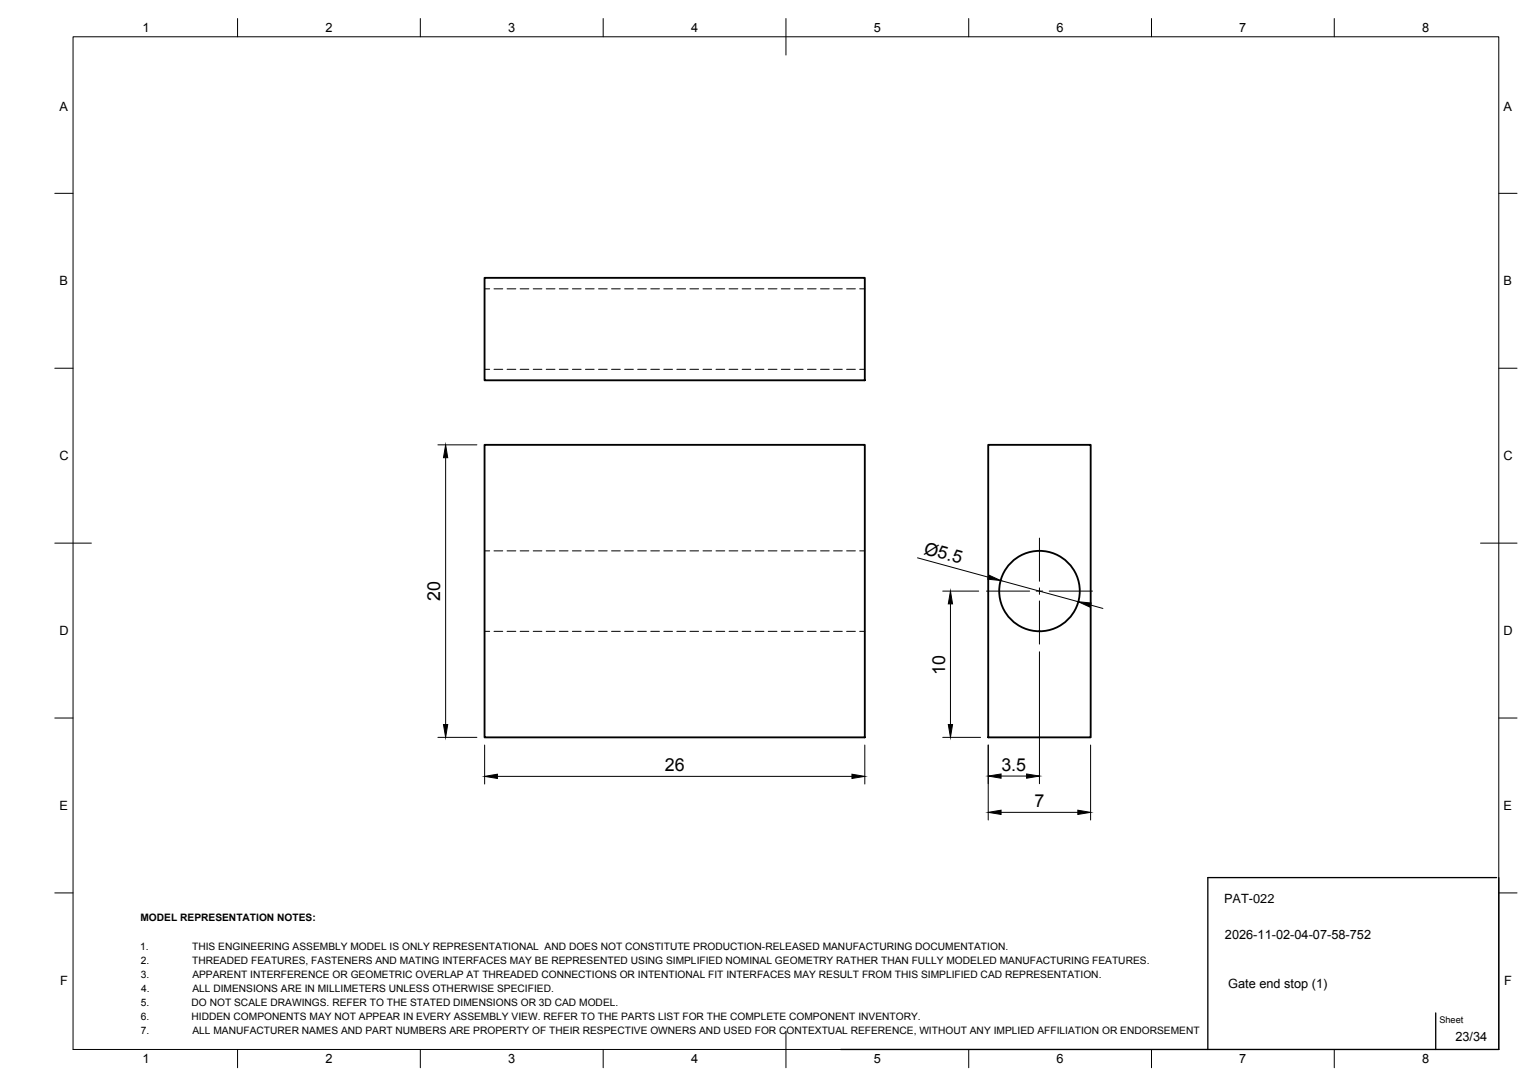
ISO-10303-21;
HEADER;
/* Generated by software containing ST-Developer
 * from STEP Tools, Inc. (www.steptools.com) 
 */

FILE_DESCRIPTION(
/* description */ ('Chute with adjustable gate'),
/* implementation_level */ '2;1');

FILE_NAME(
/* name */ 'Gate end stop (1).step',
/* time_stamp */ '2026-10-27T10:52:28-07:00',
/* author */ (''),
/* organization */ (''),
/* preprocessor_version */ 'ST-DEVELOPER v20.2',
/* originating_system */ 'Autodesk Translation Framework v15.17.0.0',
/* authorisation */ '');

FILE_SCHEMA (('AUTOMOTIVE_DESIGN { 1 0 10303 214 3 1 1 }'));
ENDSEC;

DATA;
#10=MECHANICAL_DESIGN_GEOMETRIC_PRESENTATION_REPRESENTATION('',(#432),#13094);
#368=SHAPE_REPRESENTATION_RELATIONSHIP('SRR','None',#13269,#400);
#400=ADVANCED_BREP_SHAPE_REPRESENTATION('',(#464),#13078);
#432=STYLED_ITEM('',(#13481),#464);
#464=MANIFOLD_SOLID_BREP('Body1',#7615);
#548=FACE_BOUND('',#1583,.T.);
#549=FACE_BOUND('',#1586,.T.);
#728=PLANE('',#8265);
#729=PLANE('',#8266);
#730=PLANE('',#8267);
#731=PLANE('',#8268);
#732=PLANE('',#8269);
#733=PLANE('',#8270);
#1091=FACE_OUTER_BOUND('',#1580,.T.);
#1092=FACE_OUTER_BOUND('',#1581,.T.);
#1093=FACE_OUTER_BOUND('',#1582,.T.);
#1094=FACE_OUTER_BOUND('',#1584,.T.);
#1095=FACE_OUTER_BOUND('',#1585,.T.);
#1096=FACE_OUTER_BOUND('',#1587,.T.);
#1097=FACE_OUTER_BOUND('',#1588,.T.);
#1580=EDGE_LOOP('',(#5972,#5973,#5974,#5975));
#1581=EDGE_LOOP('',(#5976,#5977,#5978,#5979));
#1582=EDGE_LOOP('',(#5980,#5981,#5982,#5983));
#1583=EDGE_LOOP('',(#5984));
#1584=EDGE_LOOP('',(#5985,#5986,#5987,#5988));
#1585=EDGE_LOOP('',(#5989,#5990,#5991,#5992));
#1586=EDGE_LOOP('',(#5993));
#1587=EDGE_LOOP('',(#5994,#5995,#5996,#5997));
#1588=EDGE_LOOP('',(#5998,#5999,#6000,#6001));
#2175=LINE('',#11756,#2952);
#2176=LINE('',#11761,#2953);
#2177=LINE('',#11763,#2954);
#2178=LINE('',#11765,#2955);
#2179=LINE('',#11766,#2956);
#2180=LINE('',#11769,#2957);
#2181=LINE('',#11771,#2958);
#2182=LINE('',#11772,#2959);
#2183=LINE('',#11775,#2960);
#2184=LINE('',#11777,#2961);
#2185=LINE('',#11778,#2962);
#2186=LINE('',#11780,#2963);
#2187=LINE('',#11781,#2964);
#2952=VECTOR('',#9569,0.274999999999999);
#2953=VECTOR('',#9574,1.);
#2954=VECTOR('',#9575,1.);
#2955=VECTOR('',#9576,1.);
#2956=VECTOR('',#9577,1.);
#2957=VECTOR('',#9580,1.);
#2958=VECTOR('',#9581,1.);
#2959=VECTOR('',#9582,1.);
#2960=VECTOR('',#9585,1.);
#2961=VECTOR('',#9586,1.);
#2962=VECTOR('',#9587,1.);
#2963=VECTOR('',#9590,1.);
#2964=VECTOR('',#9591,1.);
#3492=CIRCLE('',#8263,0.274999999999999);
#3493=CIRCLE('',#8264,0.274999999999999);
#3855=VERTEX_POINT('',#11753);
#3856=VERTEX_POINT('',#11755);
#3857=VERTEX_POINT('',#11759);
#3858=VERTEX_POINT('',#11760);
#3859=VERTEX_POINT('',#11762);
#3860=VERTEX_POINT('',#11764);
#3861=VERTEX_POINT('',#11768);
#3862=VERTEX_POINT('',#11770);
#3863=VERTEX_POINT('',#11774);
#3864=VERTEX_POINT('',#11776);
#4619=EDGE_CURVE('',#3855,#3855,#3492,.T.);
#4620=EDGE_CURVE('',#3855,#3856,#2175,.T.);
#4621=EDGE_CURVE('',#3856,#3856,#3493,.T.);
#4622=EDGE_CURVE('',#3857,#3858,#2176,.T.);
#4623=EDGE_CURVE('',#3858,#3859,#2177,.T.);
#4624=EDGE_CURVE('',#3860,#3859,#2178,.T.);
#4625=EDGE_CURVE('',#3857,#3860,#2179,.T.);
#4626=EDGE_CURVE('',#3861,#3857,#2180,.T.);
#4627=EDGE_CURVE('',#3862,#3860,#2181,.T.);
#4628=EDGE_CURVE('',#3861,#3862,#2182,.T.);
#4629=EDGE_CURVE('',#3863,#3861,#2183,.T.);
#4630=EDGE_CURVE('',#3864,#3862,#2184,.T.);
#4631=EDGE_CURVE('',#3863,#3864,#2185,.T.);
#4632=EDGE_CURVE('',#3858,#3863,#2186,.T.);
#4633=EDGE_CURVE('',#3859,#3864,#2187,.T.);
#5972=ORIENTED_EDGE('',*,*,#4619,.F.);
#5973=ORIENTED_EDGE('',*,*,#4620,.T.);
#5974=ORIENTED_EDGE('',*,*,#4621,.F.);
#5975=ORIENTED_EDGE('',*,*,#4620,.F.);
#5976=ORIENTED_EDGE('',*,*,#4622,.T.);
#5977=ORIENTED_EDGE('',*,*,#4623,.T.);
#5978=ORIENTED_EDGE('',*,*,#4624,.F.);
#5979=ORIENTED_EDGE('',*,*,#4625,.F.);
#5980=ORIENTED_EDGE('',*,*,#4626,.T.);
#5981=ORIENTED_EDGE('',*,*,#4625,.T.);
#5982=ORIENTED_EDGE('',*,*,#4627,.F.);
#5983=ORIENTED_EDGE('',*,*,#4628,.F.);
#5984=ORIENTED_EDGE('',*,*,#4621,.T.);
#5985=ORIENTED_EDGE('',*,*,#4629,.T.);
#5986=ORIENTED_EDGE('',*,*,#4628,.T.);
#5987=ORIENTED_EDGE('',*,*,#4630,.F.);
#5988=ORIENTED_EDGE('',*,*,#4631,.F.);
#5989=ORIENTED_EDGE('',*,*,#4632,.T.);
#5990=ORIENTED_EDGE('',*,*,#4631,.T.);
#5991=ORIENTED_EDGE('',*,*,#4633,.F.);
#5992=ORIENTED_EDGE('',*,*,#4623,.F.);
#5993=ORIENTED_EDGE('',*,*,#4619,.T.);
#5994=ORIENTED_EDGE('',*,*,#4633,.T.);
#5995=ORIENTED_EDGE('',*,*,#4630,.T.);
#5996=ORIENTED_EDGE('',*,*,#4627,.T.);
#5997=ORIENTED_EDGE('',*,*,#4624,.T.);
#5998=ORIENTED_EDGE('',*,*,#4632,.F.);
#5999=ORIENTED_EDGE('',*,*,#4622,.F.);
#6000=ORIENTED_EDGE('',*,*,#4626,.F.);
#6001=ORIENTED_EDGE('',*,*,#4629,.F.);
#7145=CYLINDRICAL_SURFACE('',#8262,0.274999999999999);
#7359=ADVANCED_FACE('',(#1091),#7145,.F.);
#7360=ADVANCED_FACE('',(#1092),#728,.T.);
#7361=ADVANCED_FACE('',(#1093,#548),#729,.T.);
#7362=ADVANCED_FACE('',(#1094),#730,.T.);
#7363=ADVANCED_FACE('',(#1095,#549),#731,.T.);
#7364=ADVANCED_FACE('',(#1096),#732,.T.);
#7365=ADVANCED_FACE('',(#1097),#733,.F.);
#7615=CLOSED_SHELL('',(#7359,#7360,#7361,#7362,#7363,#7364,#7365));
#8261=AXIS2_PLACEMENT_3D('',#11751,#9563,#9564);
#8262=AXIS2_PLACEMENT_3D('',#11752,#9565,#9566);
#8263=AXIS2_PLACEMENT_3D('',#11754,#9567,#9568);
#8264=AXIS2_PLACEMENT_3D('',#11757,#9570,#9571);
#8265=AXIS2_PLACEMENT_3D('',#11758,#9572,#9573);
#8266=AXIS2_PLACEMENT_3D('',#11767,#9578,#9579);
#8267=AXIS2_PLACEMENT_3D('',#11773,#9583,#9584);
#8268=AXIS2_PLACEMENT_3D('',#11779,#9588,#9589);
#8269=AXIS2_PLACEMENT_3D('',#11782,#9592,#9593);
#8270=AXIS2_PLACEMENT_3D('',#11783,#9594,#9595);
#9563=DIRECTION('axis',(0.,0.,1.));
#9564=DIRECTION('refdir',(1.,0.,0.));
#9565=DIRECTION('center_axis',(1.,0.,0.));
#9566=DIRECTION('ref_axis',(0.,0.,-1.));
#9567=DIRECTION('center_axis',(1.,0.,0.));
#9568=DIRECTION('ref_axis',(0.,0.,-1.));
#9569=DIRECTION('',(1.,0.,0.));
#9570=DIRECTION('center_axis',(-1.,0.,0.));
#9571=DIRECTION('ref_axis',(0.,0.,-1.));
#9572=DIRECTION('center_axis',(0.,1.,0.));
#9573=DIRECTION('ref_axis',(-1.,0.,0.));
#9574=DIRECTION('',(-1.,0.,0.));
#9575=DIRECTION('',(0.,0.,1.));
#9576=DIRECTION('',(-1.,0.,0.));
#9577=DIRECTION('',(0.,0.,1.));
#9578=DIRECTION('center_axis',(1.,0.,0.));
#9579=DIRECTION('ref_axis',(0.,1.,0.));
#9580=DIRECTION('',(0.,1.,0.));
#9581=DIRECTION('',(0.,1.,0.));
#9582=DIRECTION('',(0.,0.,1.));
#9583=DIRECTION('center_axis',(0.,-1.,0.));
#9584=DIRECTION('ref_axis',(1.,0.,0.));
#9585=DIRECTION('',(1.,0.,0.));
#9586=DIRECTION('',(1.,0.,0.));
#9587=DIRECTION('',(0.,0.,1.));
#9588=DIRECTION('center_axis',(-1.,0.,0.));
#9589=DIRECTION('ref_axis',(0.,-1.,0.));
#9590=DIRECTION('',(0.,-1.,0.));
#9591=DIRECTION('',(0.,-1.,0.));
#9592=DIRECTION('center_axis',(0.,0.,1.));
#9593=DIRECTION('ref_axis',(1.,0.,0.));
#9594=DIRECTION('center_axis',(0.,0.,1.));
#9595=DIRECTION('ref_axis',(1.,0.,0.));
#11751=CARTESIAN_POINT('',(0.,0.,0.));
#11752=CARTESIAN_POINT('Origin',(-1.5,11.,30.25));
#11753=CARTESIAN_POINT('',(-1.4,11.,30.525));
#11754=CARTESIAN_POINT('Origin',(-1.4,11.,30.25));
#11755=CARTESIAN_POINT('',(1.2,11.,30.525));
#11756=CARTESIAN_POINT('',(-1.5,11.,30.525));
#11757=CARTESIAN_POINT('Origin',(1.2,11.,30.25));
#11758=CARTESIAN_POINT('Origin',(1.2,12.,29.9));
#11759=CARTESIAN_POINT('',(1.2,12.,29.9));
#11760=CARTESIAN_POINT('',(-1.4,12.,29.9));
#11761=CARTESIAN_POINT('',(1.2,12.,29.9));
#11762=CARTESIAN_POINT('',(-1.4,12.,30.6));
#11763=CARTESIAN_POINT('',(-1.4,12.,29.9));
#11764=CARTESIAN_POINT('',(1.2,12.,30.6));
#11765=CARTESIAN_POINT('',(1.2,12.,30.6));
#11766=CARTESIAN_POINT('',(1.2,12.,29.9));
#11767=CARTESIAN_POINT('Origin',(1.2,10.,29.9));
#11768=CARTESIAN_POINT('',(1.2,10.,29.9));
#11769=CARTESIAN_POINT('',(1.2,10.,29.9));
#11770=CARTESIAN_POINT('',(1.2,10.,30.6));
#11771=CARTESIAN_POINT('',(1.2,10.,30.6));
#11772=CARTESIAN_POINT('',(1.2,10.,29.9));
#11773=CARTESIAN_POINT('Origin',(-1.4,10.,29.9));
#11774=CARTESIAN_POINT('',(-1.4,10.,29.9));
#11775=CARTESIAN_POINT('',(-1.4,10.,29.9));
#11776=CARTESIAN_POINT('',(-1.4,10.,30.6));
#11777=CARTESIAN_POINT('',(-1.4,10.,30.6));
#11778=CARTESIAN_POINT('',(-1.4,10.,29.9));
#11779=CARTESIAN_POINT('Origin',(-1.4,12.,29.9));
#11780=CARTESIAN_POINT('',(-1.4,12.,29.9));
#11781=CARTESIAN_POINT('',(-1.4,12.,30.6));
#11782=CARTESIAN_POINT('Origin',(-0.1,11.,30.6));
#11783=CARTESIAN_POINT('Origin',(-0.1,11.,29.9));
#13041=UNCERTAINTY_MEASURE_WITH_UNIT(LENGTH_MEASURE(0.001),#13095,
'DISTANCE_ACCURACY_VALUE',
'Maximum model space distance between geometric entities at asserted c
onnectivities');
#13057=UNCERTAINTY_MEASURE_WITH_UNIT(LENGTH_MEASURE(0.001),#13095,
'DISTANCE_ACCURACY_VALUE',
'Maximum model space distance between geometric entities at asserted c
onnectivities');
#13078=(
GEOMETRIC_REPRESENTATION_CONTEXT(3)
GLOBAL_UNCERTAINTY_ASSIGNED_CONTEXT((#13041))
GLOBAL_UNIT_ASSIGNED_CONTEXT((#13095,#13097,#13098))
REPRESENTATION_CONTEXT('','3D')
);
#13094=(
GEOMETRIC_REPRESENTATION_CONTEXT(3)
GLOBAL_UNCERTAINTY_ASSIGNED_CONTEXT((#13057))
GLOBAL_UNIT_ASSIGNED_CONTEXT((#13095,#13097,#13098))
REPRESENTATION_CONTEXT('','3D')
);
#13095=(
LENGTH_UNIT()
NAMED_UNIT(*)
SI_UNIT(.CENTI.,.METRE.)
);
#13097=(
NAMED_UNIT(*)
PLANE_ANGLE_UNIT()
SI_UNIT($,.RADIAN.)
);
#13098=(
NAMED_UNIT(*)
SI_UNIT($,.STERADIAN.)
SOLID_ANGLE_UNIT()
);
#13119=SHAPE_DEFINITION_REPRESENTATION(#13155,#13269);
#13155=PRODUCT_DEFINITION_SHAPE('',$,#13306);
#13269=SHAPE_REPRESENTATION('',(#8261),#13078);
#13285=PRODUCT_DEFINITION_CONTEXT('part definition',#13395,'design');
#13306=PRODUCT_DEFINITION('Gate end stop (1)','Gate end stop (1)',#13342,
#13285);
#13342=PRODUCT_DEFINITION_FORMATION('',$,#13417);
#13395=APPLICATION_CONTEXT(
'Core Data for Automotive Mechanical Design Process');
#13396=PRODUCT_CONTEXT('part definition',#13395,'mechanical');
#13417=PRODUCT('Gate end stop (1)','Gate end stop (1)','Gate end stop (1)',(#13396));
#13475=COLOUR_RGB('Light Blue',0.38,0.62,0.78);
#13476=FILL_AREA_STYLE_COLOUR('',#13475);
#13477=FILL_AREA_STYLE('',(#13476));
#13478=SURFACE_STYLE_FILL_AREA(#13477);
#13479=SURFACE_SIDE_STYLE('',(#13478));
#13480=SURFACE_STYLE_USAGE(.BOTH.,#13479);
#13481=PRESENTATION_STYLE_ASSIGNMENT((#13480));
ENDSEC;
END-ISO-10303-21;
